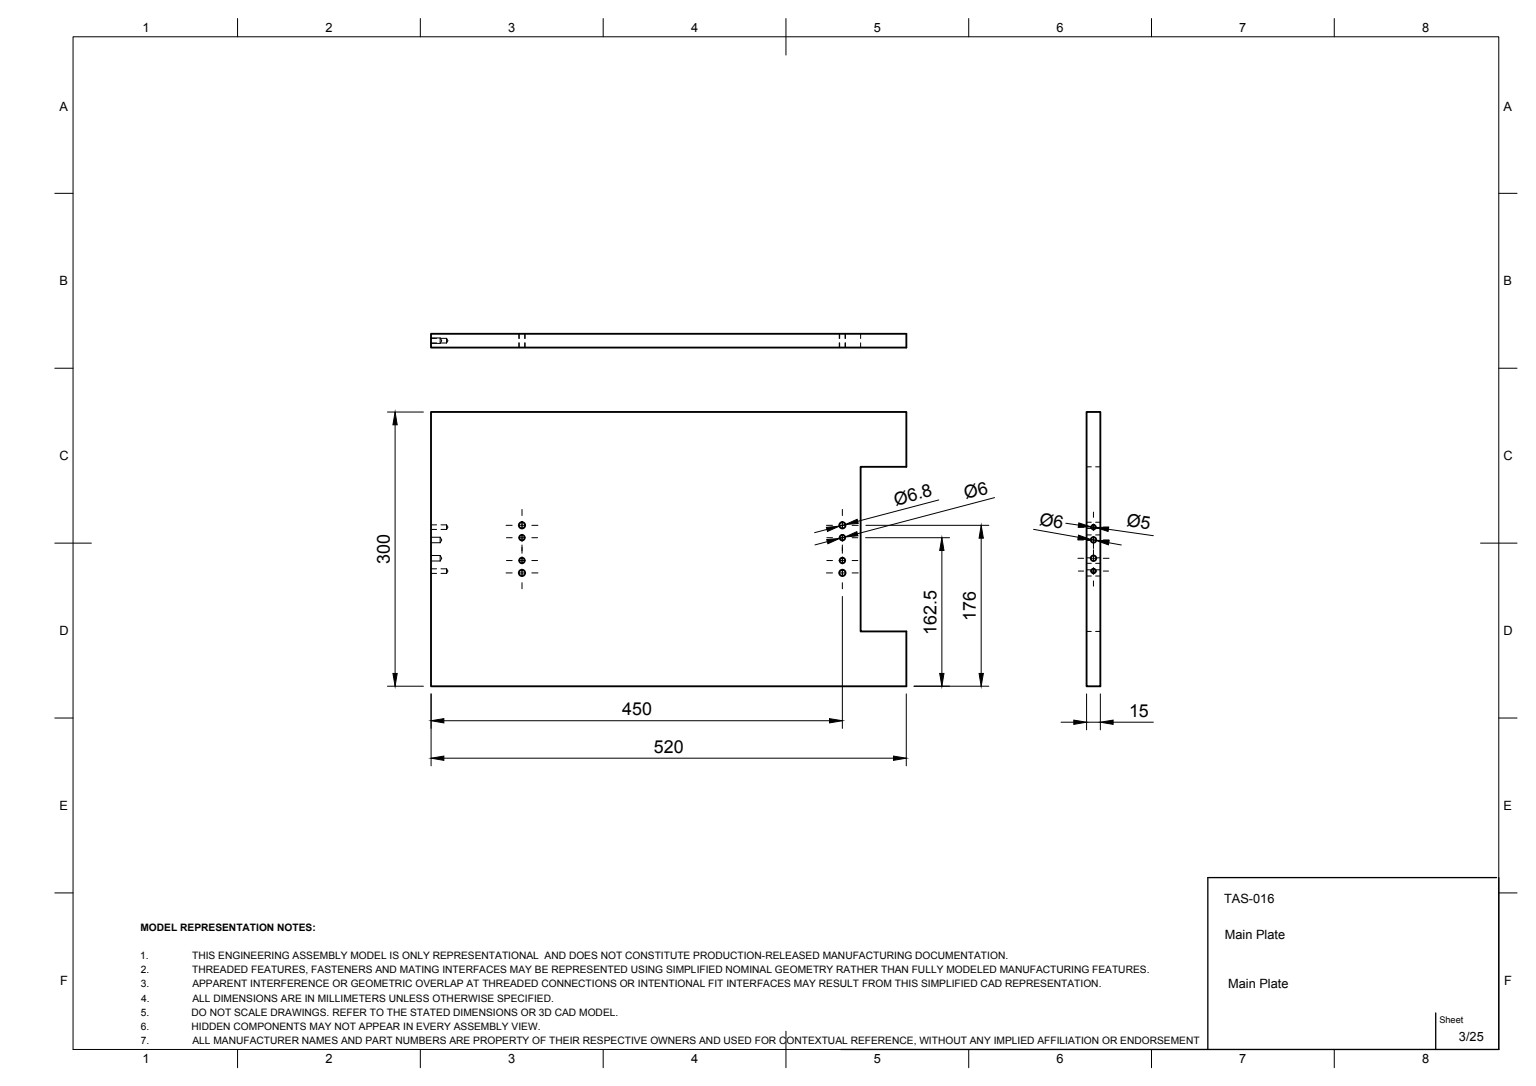
ISO-10303-21;
HEADER;
/* Generated by software containing ST-Developer
 * from STEP Tools, Inc. (www.steptools.com) 
 */

FILE_DESCRIPTION(
/* description */ ('STEP AP214'),
/* implementation_level */ '2;1');

FILE_NAME(
/* name */ 'Main Plate.step',
/* time_stamp */ '2026-11-15T14:55:55-08:00',
/* author */ (''),
/* organization */ (''),
/* preprocessor_version */ 'ST-DEVELOPER v20.2',
/* originating_system */ 'Autodesk Translation Framework v15.17.0.0',
/* authorisation */ '');

FILE_SCHEMA (('AUTOMOTIVE_DESIGN { 1 0 10303 214 3 1 1 }'));
ENDSEC;

DATA;
#10=MECHANICAL_DESIGN_GEOMETRIC_PRESENTATION_REPRESENTATION('',(#926),#57079);
#868=SHAPE_REPRESENTATION_RELATIONSHIP('SRR','None',#57250,#897);
#897=ADVANCED_BREP_SHAPE_REPRESENTATION('',(#963),#57042);
#926=STYLED_ITEM('',(#57444),#963);
#963=MANIFOLD_SOLID_BREP('Body1',#24526);
#1000=FACE_BOUND('',#3553,.T.);
#1001=FACE_BOUND('',#3554,.T.);
#1002=FACE_BOUND('',#3555,.T.);
#1003=FACE_BOUND('',#3556,.T.);
#1004=FACE_BOUND('',#3560,.T.);
#1005=FACE_BOUND('',#3561,.T.);
#1006=FACE_BOUND('',#3562,.T.);
#1007=FACE_BOUND('',#3563,.T.);
#1008=FACE_BOUND('',#3564,.T.);
#1009=FACE_BOUND('',#3565,.T.);
#1010=FACE_BOUND('',#3566,.T.);
#1011=FACE_BOUND('',#3567,.T.);
#1012=FACE_BOUND('',#3569,.T.);
#1013=FACE_BOUND('',#3570,.T.);
#1014=FACE_BOUND('',#3571,.T.);
#1015=FACE_BOUND('',#3572,.T.);
#1016=FACE_BOUND('',#3573,.T.);
#1017=FACE_BOUND('',#3574,.T.);
#1018=FACE_BOUND('',#3575,.T.);
#1019=FACE_BOUND('',#3576,.T.);
#1342=PLANE('',#24925);
#1343=PLANE('',#24926);
#1344=PLANE('',#24927);
#1345=PLANE('',#24928);
#1346=PLANE('',#24929);
#1347=PLANE('',#24930);
#1348=PLANE('',#24931);
#1349=PLANE('',#24932);
#1350=PLANE('',#24933);
#1351=PLANE('',#24934);
#2105=CONICAL_SURFACE('',#24912,3.,1.02974425867665);
#2106=CONICAL_SURFACE('',#24916,3.,1.02974425867665);
#2107=CONICAL_SURFACE('',#24920,2.49999999999999,1.02974425867666);
#2108=CONICAL_SURFACE('',#24924,2.49999999999999,1.02974425867666);
#2159=FACE_OUTER_BOUND('',#3534,.T.);
#2160=FACE_OUTER_BOUND('',#3535,.T.);
#2161=FACE_OUTER_BOUND('',#3536,.T.);
#2162=FACE_OUTER_BOUND('',#3537,.T.);
#2163=FACE_OUTER_BOUND('',#3538,.T.);
#2164=FACE_OUTER_BOUND('',#3539,.T.);
#2165=FACE_OUTER_BOUND('',#3540,.T.);
#2166=FACE_OUTER_BOUND('',#3541,.T.);
#2167=FACE_OUTER_BOUND('',#3542,.T.);
#2168=FACE_OUTER_BOUND('',#3543,.T.);
#2169=FACE_OUTER_BOUND('',#3544,.T.);
#2170=FACE_OUTER_BOUND('',#3545,.T.);
#2171=FACE_OUTER_BOUND('',#3546,.T.);
#2172=FACE_OUTER_BOUND('',#3547,.T.);
#2173=FACE_OUTER_BOUND('',#3548,.T.);
#2174=FACE_OUTER_BOUND('',#3549,.T.);
#2175=FACE_OUTER_BOUND('',#3550,.T.);
#2176=FACE_OUTER_BOUND('',#3551,.T.);
#2177=FACE_OUTER_BOUND('',#3552,.T.);
#2178=FACE_OUTER_BOUND('',#3557,.T.);
#2179=FACE_OUTER_BOUND('',#3558,.T.);
#2180=FACE_OUTER_BOUND('',#3559,.T.);
#2181=FACE_OUTER_BOUND('',#3568,.T.);
#2182=FACE_OUTER_BOUND('',#3577,.T.);
#2183=FACE_OUTER_BOUND('',#3578,.T.);
#2184=FACE_OUTER_BOUND('',#3579,.T.);
#3534=EDGE_LOOP('',(#15916,#15917,#15918,#15919));
#3535=EDGE_LOOP('',(#15920,#15921,#15922,#15923));
#3536=EDGE_LOOP('',(#15924,#15925,#15926,#15927));
#3537=EDGE_LOOP('',(#15928,#15929,#15930,#15931));
#3538=EDGE_LOOP('',(#15932,#15933,#15934,#15935));
#3539=EDGE_LOOP('',(#15936,#15937,#15938,#15939));
#3540=EDGE_LOOP('',(#15940,#15941,#15942,#15943));
#3541=EDGE_LOOP('',(#15944,#15945,#15946,#15947));
#3542=EDGE_LOOP('',(#15948,#15949,#15950,#15951));
#3543=EDGE_LOOP('',(#15952,#15953,#15954));
#3544=EDGE_LOOP('',(#15955,#15956,#15957,#15958));
#3545=EDGE_LOOP('',(#15959,#15960,#15961));
#3546=EDGE_LOOP('',(#15962,#15963,#15964,#15965));
#3547=EDGE_LOOP('',(#15966,#15967,#15968));
#3548=EDGE_LOOP('',(#15969,#15970,#15971,#15972));
#3549=EDGE_LOOP('',(#15973,#15974,#15975));
#3550=EDGE_LOOP('',(#15976,#15977,#15978,#15979));
#3551=EDGE_LOOP('',(#15980,#15981,#15982,#15983));
#3552=EDGE_LOOP('',(#15984,#15985,#15986,#15987));
#3553=EDGE_LOOP('',(#15988));
#3554=EDGE_LOOP('',(#15989));
#3555=EDGE_LOOP('',(#15990));
#3556=EDGE_LOOP('',(#15991));
#3557=EDGE_LOOP('',(#15992,#15993,#15994,#15995));
#3558=EDGE_LOOP('',(#15996,#15997,#15998,#15999));
#3559=EDGE_LOOP('',(#16000,#16001,#16002,#16003,#16004,#16005,#16006,#16007));
#3560=EDGE_LOOP('',(#16008));
#3561=EDGE_LOOP('',(#16009));
#3562=EDGE_LOOP('',(#16010));
#3563=EDGE_LOOP('',(#16011));
#3564=EDGE_LOOP('',(#16012));
#3565=EDGE_LOOP('',(#16013));
#3566=EDGE_LOOP('',(#16014));
#3567=EDGE_LOOP('',(#16015));
#3568=EDGE_LOOP('',(#16016,#16017,#16018,#16019,#16020,#16021,#16022,#16023));
#3569=EDGE_LOOP('',(#16024));
#3570=EDGE_LOOP('',(#16025));
#3571=EDGE_LOOP('',(#16026));
#3572=EDGE_LOOP('',(#16027));
#3573=EDGE_LOOP('',(#16028));
#3574=EDGE_LOOP('',(#16029));
#3575=EDGE_LOOP('',(#16030));
#3576=EDGE_LOOP('',(#16031));
#3577=EDGE_LOOP('',(#16032,#16033,#16034,#16035));
#3578=EDGE_LOOP('',(#16036,#16037,#16038,#16039));
#3579=EDGE_LOOP('',(#16040,#16041,#16042,#16043));
#5251=LINE('',#34638,#7218);
#5252=LINE('',#34644,#7219);
#5253=LINE('',#34650,#7220);
#5254=LINE('',#34656,#7221);
#5255=LINE('',#34662,#7222);
#5256=LINE('',#34668,#7223);
#5257=LINE('',#34674,#7224);
#5258=LINE('',#34680,#7225);
#5259=LINE('',#34686,#7226);
#5260=LINE('',#34690,#7227);
#5261=LINE('',#34695,#7228);
#5262=LINE('',#34699,#7229);
#5263=LINE('',#34704,#7230);
#5264=LINE('',#34708,#7231);
#5265=LINE('',#34713,#7232);
#5266=LINE('',#34717,#7233);
#5267=LINE('',#34721,#7234);
#5268=LINE('',#34723,#7235);
#5269=LINE('',#34725,#7236);
#5270=LINE('',#34726,#7237);
#5271=LINE('',#34730,#7238);
#5272=LINE('',#34732,#7239);
#5273=LINE('',#34734,#7240);
#5274=LINE('',#34735,#7241);
#5275=LINE('',#34738,#7242);
#5276=LINE('',#34740,#7243);
#5277=LINE('',#34741,#7244);
#5278=LINE('',#34743,#7245);
#5279=LINE('',#34744,#7246);
#5280=LINE('',#34747,#7247);
#5281=LINE('',#34749,#7248);
#5282=LINE('',#34750,#7249);
#5283=LINE('',#34753,#7250);
#5284=LINE('',#34755,#7251);
#5285=LINE('',#34756,#7252);
#5286=LINE('',#34759,#7253);
#5287=LINE('',#34761,#7254);
#5288=LINE('',#34762,#7255);
#5289=LINE('',#34764,#7256);
#5290=LINE('',#34766,#7257);
#7218=VECTOR('',#27485,3.);
#7219=VECTOR('',#27492,3.);
#7220=VECTOR('',#27499,3.);
#7221=VECTOR('',#27506,3.);
#7222=VECTOR('',#27513,3.4);
#7223=VECTOR('',#27520,3.4);
#7224=VECTOR('',#27527,3.4);
#7225=VECTOR('',#27534,3.4);
#7226=VECTOR('',#27541,3.);
#7227=VECTOR('',#27546,3.);
#7228=VECTOR('',#27551,3.);
#7229=VECTOR('',#27556,3.);
#7230=VECTOR('',#27561,2.49999999999999);
#7231=VECTOR('',#27566,2.49999999999999);
#7232=VECTOR('',#27571,2.49999999999999);
#7233=VECTOR('',#27576,2.49999999999999);
#7234=VECTOR('',#27579,1000.);
#7235=VECTOR('',#27580,1000.);
#7236=VECTOR('',#27581,1000.);
#7237=VECTOR('',#27582,1000.);
#7238=VECTOR('',#27585,1000.);
#7239=VECTOR('',#27586,1000.);
#7240=VECTOR('',#27587,1000.);
#7241=VECTOR('',#27588,1000.);
#7242=VECTOR('',#27591,1000.);
#7243=VECTOR('',#27592,1000.);
#7244=VECTOR('',#27593,1000.);
#7245=VECTOR('',#27596,1000.);
#7246=VECTOR('',#27597,1000.);
#7247=VECTOR('',#27600,1000.);
#7248=VECTOR('',#27601,1000.);
#7249=VECTOR('',#27602,1000.);
#7250=VECTOR('',#27605,1000.);
#7251=VECTOR('',#27606,1000.);
#7252=VECTOR('',#27607,1000.);
#7253=VECTOR('',#27610,1000.);
#7254=VECTOR('',#27611,1000.);
#7255=VECTOR('',#27612,1000.);
#7256=VECTOR('',#27615,1000.);
#7257=VECTOR('',#27618,1000.);
#9185=CIRCLE('',#24886,3.);
#9186=CIRCLE('',#24887,3.);
#9187=CIRCLE('',#24889,3.);
#9188=CIRCLE('',#24890,3.);
#9189=CIRCLE('',#24892,3.);
#9190=CIRCLE('',#24893,3.);
#9191=CIRCLE('',#24895,3.);
#9192=CIRCLE('',#24896,3.);
#9193=CIRCLE('',#24898,3.4);
#9194=CIRCLE('',#24899,3.4);
#9195=CIRCLE('',#24901,3.4);
#9196=CIRCLE('',#24902,3.4);
#9197=CIRCLE('',#24904,3.4);
#9198=CIRCLE('',#24905,3.4);
#9199=CIRCLE('',#24907,3.4);
#9200=CIRCLE('',#24908,3.4);
#9201=CIRCLE('',#24910,3.);
#9202=CIRCLE('',#24911,3.);
#9203=CIRCLE('',#24914,3.);
#9204=CIRCLE('',#24915,3.);
#9205=CIRCLE('',#24918,2.49999999999999);
#9206=CIRCLE('',#24919,2.49999999999999);
#9207=CIRCLE('',#24922,2.49999999999999);
#9208=CIRCLE('',#24923,2.49999999999999);
#10279=VERTEX_POINT('',#34635);
#10280=VERTEX_POINT('',#34637);
#10281=VERTEX_POINT('',#34641);
#10282=VERTEX_POINT('',#34643);
#10283=VERTEX_POINT('',#34647);
#10284=VERTEX_POINT('',#34649);
#10285=VERTEX_POINT('',#34653);
#10286=VERTEX_POINT('',#34655);
#10287=VERTEX_POINT('',#34659);
#10288=VERTEX_POINT('',#34661);
#10289=VERTEX_POINT('',#34665);
#10290=VERTEX_POINT('',#34667);
#10291=VERTEX_POINT('',#34671);
#10292=VERTEX_POINT('',#34673);
#10293=VERTEX_POINT('',#34677);
#10294=VERTEX_POINT('',#34679);
#10295=VERTEX_POINT('',#34683);
#10296=VERTEX_POINT('',#34685);
#10297=VERTEX_POINT('',#34689);
#10298=VERTEX_POINT('',#34692);
#10299=VERTEX_POINT('',#34694);
#10300=VERTEX_POINT('',#34698);
#10301=VERTEX_POINT('',#34701);
#10302=VERTEX_POINT('',#34703);
#10303=VERTEX_POINT('',#34707);
#10304=VERTEX_POINT('',#34710);
#10305=VERTEX_POINT('',#34712);
#10306=VERTEX_POINT('',#34716);
#10307=VERTEX_POINT('',#34719);
#10308=VERTEX_POINT('',#34720);
#10309=VERTEX_POINT('',#34722);
#10310=VERTEX_POINT('',#34724);
#10311=VERTEX_POINT('',#34728);
#10312=VERTEX_POINT('',#34729);
#10313=VERTEX_POINT('',#34731);
#10314=VERTEX_POINT('',#34733);
#10315=VERTEX_POINT('',#34737);
#10316=VERTEX_POINT('',#34739);
#10317=VERTEX_POINT('',#34746);
#10318=VERTEX_POINT('',#34748);
#10319=VERTEX_POINT('',#34752);
#10320=VERTEX_POINT('',#34754);
#10321=VERTEX_POINT('',#34758);
#10322=VERTEX_POINT('',#34760);
#12503=EDGE_CURVE('',#10279,#10279,#9185,.T.);
#12504=EDGE_CURVE('',#10279,#10280,#5251,.T.);
#12505=EDGE_CURVE('',#10280,#10280,#9186,.T.);
#12506=EDGE_CURVE('',#10281,#10281,#9187,.T.);
#12507=EDGE_CURVE('',#10281,#10282,#5252,.T.);
#12508=EDGE_CURVE('',#10282,#10282,#9188,.T.);
#12509=EDGE_CURVE('',#10283,#10283,#9189,.T.);
#12510=EDGE_CURVE('',#10283,#10284,#5253,.T.);
#12511=EDGE_CURVE('',#10284,#10284,#9190,.T.);
#12512=EDGE_CURVE('',#10285,#10285,#9191,.T.);
#12513=EDGE_CURVE('',#10285,#10286,#5254,.T.);
#12514=EDGE_CURVE('',#10286,#10286,#9192,.T.);
#12515=EDGE_CURVE('',#10287,#10287,#9193,.T.);
#12516=EDGE_CURVE('',#10287,#10288,#5255,.T.);
#12517=EDGE_CURVE('',#10288,#10288,#9194,.T.);
#12518=EDGE_CURVE('',#10289,#10289,#9195,.T.);
#12519=EDGE_CURVE('',#10289,#10290,#5256,.T.);
#12520=EDGE_CURVE('',#10290,#10290,#9196,.T.);
#12521=EDGE_CURVE('',#10291,#10291,#9197,.T.);
#12522=EDGE_CURVE('',#10291,#10292,#5257,.T.);
#12523=EDGE_CURVE('',#10292,#10292,#9198,.T.);
#12524=EDGE_CURVE('',#10293,#10293,#9199,.T.);
#12525=EDGE_CURVE('',#10293,#10294,#5258,.T.);
#12526=EDGE_CURVE('',#10294,#10294,#9200,.T.);
#12527=EDGE_CURVE('',#10295,#10295,#9201,.T.);
#12528=EDGE_CURVE('',#10295,#10296,#5259,.T.);
#12529=EDGE_CURVE('',#10296,#10296,#9202,.T.);
#12530=EDGE_CURVE('',#10297,#10295,#5260,.T.);
#12531=EDGE_CURVE('',#10298,#10298,#9203,.T.);
#12532=EDGE_CURVE('',#10298,#10299,#5261,.T.);
#12533=EDGE_CURVE('',#10299,#10299,#9204,.T.);
#12534=EDGE_CURVE('',#10300,#10298,#5262,.T.);
#12535=EDGE_CURVE('',#10301,#10301,#9205,.T.);
#12536=EDGE_CURVE('',#10301,#10302,#5263,.T.);
#12537=EDGE_CURVE('',#10302,#10302,#9206,.T.);
#12538=EDGE_CURVE('',#10303,#10301,#5264,.T.);
#12539=EDGE_CURVE('',#10304,#10304,#9207,.T.);
#12540=EDGE_CURVE('',#10304,#10305,#5265,.T.);
#12541=EDGE_CURVE('',#10305,#10305,#9208,.T.);
#12542=EDGE_CURVE('',#10306,#10304,#5266,.T.);
#12543=EDGE_CURVE('',#10307,#10308,#5267,.T.);
#12544=EDGE_CURVE('',#10308,#10309,#5268,.T.);
#12545=EDGE_CURVE('',#10310,#10309,#5269,.T.);
#12546=EDGE_CURVE('',#10310,#10307,#5270,.T.);
#12547=EDGE_CURVE('',#10311,#10312,#5271,.T.);
#12548=EDGE_CURVE('',#10313,#10312,#5272,.T.);
#12549=EDGE_CURVE('',#10314,#10313,#5273,.T.);
#12550=EDGE_CURVE('',#10314,#10311,#5274,.T.);
#12551=EDGE_CURVE('',#10312,#10315,#5275,.T.);
#12552=EDGE_CURVE('',#10316,#10315,#5276,.T.);
#12553=EDGE_CURVE('',#10313,#10316,#5277,.T.);
#12554=EDGE_CURVE('',#10315,#10307,#5278,.T.);
#12555=EDGE_CURVE('',#10316,#10310,#5279,.T.);
#12556=EDGE_CURVE('',#10317,#10314,#5280,.T.);
#12557=EDGE_CURVE('',#10318,#10317,#5281,.T.);
#12558=EDGE_CURVE('',#10318,#10311,#5282,.T.);
#12559=EDGE_CURVE('',#10319,#10309,#5283,.T.);
#12560=EDGE_CURVE('',#10320,#10319,#5284,.T.);
#12561=EDGE_CURVE('',#10317,#10320,#5285,.T.);
#12562=EDGE_CURVE('',#10321,#10308,#5286,.T.);
#12563=EDGE_CURVE('',#10318,#10322,#5287,.T.);
#12564=EDGE_CURVE('',#10322,#10321,#5288,.T.);
#12565=EDGE_CURVE('',#10321,#10319,#5289,.T.);
#12566=EDGE_CURVE('',#10322,#10320,#5290,.T.);
#15916=ORIENTED_EDGE('',*,*,#12503,.F.);
#15917=ORIENTED_EDGE('',*,*,#12504,.T.);
#15918=ORIENTED_EDGE('',*,*,#12505,.T.);
#15919=ORIENTED_EDGE('',*,*,#12504,.F.);
#15920=ORIENTED_EDGE('',*,*,#12506,.F.);
#15921=ORIENTED_EDGE('',*,*,#12507,.T.);
#15922=ORIENTED_EDGE('',*,*,#12508,.T.);
#15923=ORIENTED_EDGE('',*,*,#12507,.F.);
#15924=ORIENTED_EDGE('',*,*,#12509,.F.);
#15925=ORIENTED_EDGE('',*,*,#12510,.T.);
#15926=ORIENTED_EDGE('',*,*,#12511,.T.);
#15927=ORIENTED_EDGE('',*,*,#12510,.F.);
#15928=ORIENTED_EDGE('',*,*,#12512,.F.);
#15929=ORIENTED_EDGE('',*,*,#12513,.T.);
#15930=ORIENTED_EDGE('',*,*,#12514,.T.);
#15931=ORIENTED_EDGE('',*,*,#12513,.F.);
#15932=ORIENTED_EDGE('',*,*,#12515,.F.);
#15933=ORIENTED_EDGE('',*,*,#12516,.T.);
#15934=ORIENTED_EDGE('',*,*,#12517,.T.);
#15935=ORIENTED_EDGE('',*,*,#12516,.F.);
#15936=ORIENTED_EDGE('',*,*,#12518,.F.);
#15937=ORIENTED_EDGE('',*,*,#12519,.T.);
#15938=ORIENTED_EDGE('',*,*,#12520,.T.);
#15939=ORIENTED_EDGE('',*,*,#12519,.F.);
#15940=ORIENTED_EDGE('',*,*,#12521,.F.);
#15941=ORIENTED_EDGE('',*,*,#12522,.T.);
#15942=ORIENTED_EDGE('',*,*,#12523,.T.);
#15943=ORIENTED_EDGE('',*,*,#12522,.F.);
#15944=ORIENTED_EDGE('',*,*,#12524,.F.);
#15945=ORIENTED_EDGE('',*,*,#12525,.T.);
#15946=ORIENTED_EDGE('',*,*,#12526,.T.);
#15947=ORIENTED_EDGE('',*,*,#12525,.F.);
#15948=ORIENTED_EDGE('',*,*,#12527,.F.);
#15949=ORIENTED_EDGE('',*,*,#12528,.T.);
#15950=ORIENTED_EDGE('',*,*,#12529,.T.);
#15951=ORIENTED_EDGE('',*,*,#12528,.F.);
#15952=ORIENTED_EDGE('',*,*,#12530,.T.);
#15953=ORIENTED_EDGE('',*,*,#12527,.T.);
#15954=ORIENTED_EDGE('',*,*,#12530,.F.);
#15955=ORIENTED_EDGE('',*,*,#12531,.F.);
#15956=ORIENTED_EDGE('',*,*,#12532,.T.);
#15957=ORIENTED_EDGE('',*,*,#12533,.T.);
#15958=ORIENTED_EDGE('',*,*,#12532,.F.);
#15959=ORIENTED_EDGE('',*,*,#12534,.T.);
#15960=ORIENTED_EDGE('',*,*,#12531,.T.);
#15961=ORIENTED_EDGE('',*,*,#12534,.F.);
#15962=ORIENTED_EDGE('',*,*,#12535,.F.);
#15963=ORIENTED_EDGE('',*,*,#12536,.T.);
#15964=ORIENTED_EDGE('',*,*,#12537,.T.);
#15965=ORIENTED_EDGE('',*,*,#12536,.F.);
#15966=ORIENTED_EDGE('',*,*,#12538,.T.);
#15967=ORIENTED_EDGE('',*,*,#12535,.T.);
#15968=ORIENTED_EDGE('',*,*,#12538,.F.);
#15969=ORIENTED_EDGE('',*,*,#12539,.F.);
#15970=ORIENTED_EDGE('',*,*,#12540,.T.);
#15971=ORIENTED_EDGE('',*,*,#12541,.T.);
#15972=ORIENTED_EDGE('',*,*,#12540,.F.);
#15973=ORIENTED_EDGE('',*,*,#12542,.T.);
#15974=ORIENTED_EDGE('',*,*,#12539,.T.);
#15975=ORIENTED_EDGE('',*,*,#12542,.F.);
#15976=ORIENTED_EDGE('',*,*,#12543,.T.);
#15977=ORIENTED_EDGE('',*,*,#12544,.T.);
#15978=ORIENTED_EDGE('',*,*,#12545,.F.);
#15979=ORIENTED_EDGE('',*,*,#12546,.T.);
#15980=ORIENTED_EDGE('',*,*,#12547,.T.);
#15981=ORIENTED_EDGE('',*,*,#12548,.F.);
#15982=ORIENTED_EDGE('',*,*,#12549,.F.);
#15983=ORIENTED_EDGE('',*,*,#12550,.T.);
#15984=ORIENTED_EDGE('',*,*,#12551,.T.);
#15985=ORIENTED_EDGE('',*,*,#12552,.F.);
#15986=ORIENTED_EDGE('',*,*,#12553,.F.);
#15987=ORIENTED_EDGE('',*,*,#12548,.T.);
#15988=ORIENTED_EDGE('',*,*,#12529,.F.);
#15989=ORIENTED_EDGE('',*,*,#12533,.F.);
#15990=ORIENTED_EDGE('',*,*,#12537,.F.);
#15991=ORIENTED_EDGE('',*,*,#12541,.F.);
#15992=ORIENTED_EDGE('',*,*,#12554,.T.);
#15993=ORIENTED_EDGE('',*,*,#12546,.F.);
#15994=ORIENTED_EDGE('',*,*,#12555,.F.);
#15995=ORIENTED_EDGE('',*,*,#12552,.T.);
#15996=ORIENTED_EDGE('',*,*,#12556,.F.);
#15997=ORIENTED_EDGE('',*,*,#12557,.F.);
#15998=ORIENTED_EDGE('',*,*,#12558,.T.);
#15999=ORIENTED_EDGE('',*,*,#12550,.F.);
#16000=ORIENTED_EDGE('',*,*,#12545,.T.);
#16001=ORIENTED_EDGE('',*,*,#12559,.F.);
#16002=ORIENTED_EDGE('',*,*,#12560,.F.);
#16003=ORIENTED_EDGE('',*,*,#12561,.F.);
#16004=ORIENTED_EDGE('',*,*,#12556,.T.);
#16005=ORIENTED_EDGE('',*,*,#12549,.T.);
#16006=ORIENTED_EDGE('',*,*,#12553,.T.);
#16007=ORIENTED_EDGE('',*,*,#12555,.T.);
#16008=ORIENTED_EDGE('',*,*,#12505,.F.);
#16009=ORIENTED_EDGE('',*,*,#12508,.F.);
#16010=ORIENTED_EDGE('',*,*,#12511,.F.);
#16011=ORIENTED_EDGE('',*,*,#12514,.F.);
#16012=ORIENTED_EDGE('',*,*,#12517,.F.);
#16013=ORIENTED_EDGE('',*,*,#12520,.F.);
#16014=ORIENTED_EDGE('',*,*,#12523,.F.);
#16015=ORIENTED_EDGE('',*,*,#12526,.F.);
#16016=ORIENTED_EDGE('',*,*,#12562,.T.);
#16017=ORIENTED_EDGE('',*,*,#12543,.F.);
#16018=ORIENTED_EDGE('',*,*,#12554,.F.);
#16019=ORIENTED_EDGE('',*,*,#12551,.F.);
#16020=ORIENTED_EDGE('',*,*,#12547,.F.);
#16021=ORIENTED_EDGE('',*,*,#12558,.F.);
#16022=ORIENTED_EDGE('',*,*,#12563,.T.);
#16023=ORIENTED_EDGE('',*,*,#12564,.T.);
#16024=ORIENTED_EDGE('',*,*,#12503,.T.);
#16025=ORIENTED_EDGE('',*,*,#12506,.T.);
#16026=ORIENTED_EDGE('',*,*,#12509,.T.);
#16027=ORIENTED_EDGE('',*,*,#12512,.T.);
#16028=ORIENTED_EDGE('',*,*,#12515,.T.);
#16029=ORIENTED_EDGE('',*,*,#12518,.T.);
#16030=ORIENTED_EDGE('',*,*,#12521,.T.);
#16031=ORIENTED_EDGE('',*,*,#12524,.T.);
#16032=ORIENTED_EDGE('',*,*,#12559,.T.);
#16033=ORIENTED_EDGE('',*,*,#12544,.F.);
#16034=ORIENTED_EDGE('',*,*,#12562,.F.);
#16035=ORIENTED_EDGE('',*,*,#12565,.T.);
#16036=ORIENTED_EDGE('',*,*,#12560,.T.);
#16037=ORIENTED_EDGE('',*,*,#12565,.F.);
#16038=ORIENTED_EDGE('',*,*,#12564,.F.);
#16039=ORIENTED_EDGE('',*,*,#12566,.T.);
#16040=ORIENTED_EDGE('',*,*,#12561,.T.);
#16041=ORIENTED_EDGE('',*,*,#12566,.F.);
#16042=ORIENTED_EDGE('',*,*,#12563,.F.);
#16043=ORIENTED_EDGE('',*,*,#12557,.T.);
#22742=CYLINDRICAL_SURFACE('',#24885,3.);
#22743=CYLINDRICAL_SURFACE('',#24888,3.);
#22744=CYLINDRICAL_SURFACE('',#24891,3.);
#22745=CYLINDRICAL_SURFACE('',#24894,3.);
#22746=CYLINDRICAL_SURFACE('',#24897,3.4);
#22747=CYLINDRICAL_SURFACE('',#24900,3.4);
#22748=CYLINDRICAL_SURFACE('',#24903,3.4);
#22749=CYLINDRICAL_SURFACE('',#24906,3.4);
#22750=CYLINDRICAL_SURFACE('',#24909,3.);
#22751=CYLINDRICAL_SURFACE('',#24913,3.);
#22752=CYLINDRICAL_SURFACE('',#24917,2.49999999999999);
#22753=CYLINDRICAL_SURFACE('',#24921,2.49999999999999);
#23151=ADVANCED_FACE('',(#2159),#22742,.F.);
#23152=ADVANCED_FACE('',(#2160),#22743,.F.);
#23153=ADVANCED_FACE('',(#2161),#22744,.F.);
#23154=ADVANCED_FACE('',(#2162),#22745,.F.);
#23155=ADVANCED_FACE('',(#2163),#22746,.F.);
#23156=ADVANCED_FACE('',(#2164),#22747,.F.);
#23157=ADVANCED_FACE('',(#2165),#22748,.F.);
#23158=ADVANCED_FACE('',(#2166),#22749,.F.);
#23159=ADVANCED_FACE('',(#2167),#22750,.F.);
#23160=ADVANCED_FACE('',(#2168),#2105,.F.);
#23161=ADVANCED_FACE('',(#2169),#22751,.F.);
#23162=ADVANCED_FACE('',(#2170),#2106,.F.);
#23163=ADVANCED_FACE('',(#2171),#22752,.F.);
#23164=ADVANCED_FACE('',(#2172),#2107,.F.);
#23165=ADVANCED_FACE('',(#2173),#22753,.F.);
#23166=ADVANCED_FACE('',(#2174),#2108,.F.);
#23167=ADVANCED_FACE('',(#2175),#1342,.F.);
#23168=ADVANCED_FACE('',(#2176),#1343,.F.);
#23169=ADVANCED_FACE('',(#2177,#1000,#1001,#1002,#1003),#1344,.F.);
#23170=ADVANCED_FACE('',(#2178),#1345,.F.);
#23171=ADVANCED_FACE('',(#2179),#1346,.F.);
#23172=ADVANCED_FACE('',(#2180,#1004,#1005,#1006,#1007,#1008,#1009,#1010,
#1011),#1347,.F.);
#23173=ADVANCED_FACE('',(#2181,#1012,#1013,#1014,#1015,#1016,#1017,#1018,
#1019),#1348,.T.);
#23174=ADVANCED_FACE('',(#2182),#1349,.F.);
#23175=ADVANCED_FACE('',(#2183),#1350,.F.);
#23176=ADVANCED_FACE('',(#2184),#1351,.F.);
#24526=CLOSED_SHELL('',(#23151,#23152,#23153,#23154,#23155,#23156,#23157,
#23158,#23159,#23160,#23161,#23162,#23163,#23164,#23165,#23166,#23167,#23168,
#23169,#23170,#23171,#23172,#23173,#23174,#23175,#23176));
#24884=AXIS2_PLACEMENT_3D('',#34633,#27479,#27480);
#24885=AXIS2_PLACEMENT_3D('',#34634,#27481,#27482);
#24886=AXIS2_PLACEMENT_3D('',#34636,#27483,#27484);
#24887=AXIS2_PLACEMENT_3D('',#34639,#27486,#27487);
#24888=AXIS2_PLACEMENT_3D('',#34640,#27488,#27489);
#24889=AXIS2_PLACEMENT_3D('',#34642,#27490,#27491);
#24890=AXIS2_PLACEMENT_3D('',#34645,#27493,#27494);
#24891=AXIS2_PLACEMENT_3D('',#34646,#27495,#27496);
#24892=AXIS2_PLACEMENT_3D('',#34648,#27497,#27498);
#24893=AXIS2_PLACEMENT_3D('',#34651,#27500,#27501);
#24894=AXIS2_PLACEMENT_3D('',#34652,#27502,#27503);
#24895=AXIS2_PLACEMENT_3D('',#34654,#27504,#27505);
#24896=AXIS2_PLACEMENT_3D('',#34657,#27507,#27508);
#24897=AXIS2_PLACEMENT_3D('',#34658,#27509,#27510);
#24898=AXIS2_PLACEMENT_3D('',#34660,#27511,#27512);
#24899=AXIS2_PLACEMENT_3D('',#34663,#27514,#27515);
#24900=AXIS2_PLACEMENT_3D('',#34664,#27516,#27517);
#24901=AXIS2_PLACEMENT_3D('',#34666,#27518,#27519);
#24902=AXIS2_PLACEMENT_3D('',#34669,#27521,#27522);
#24903=AXIS2_PLACEMENT_3D('',#34670,#27523,#27524);
#24904=AXIS2_PLACEMENT_3D('',#34672,#27525,#27526);
#24905=AXIS2_PLACEMENT_3D('',#34675,#27528,#27529);
#24906=AXIS2_PLACEMENT_3D('',#34676,#27530,#27531);
#24907=AXIS2_PLACEMENT_3D('',#34678,#27532,#27533);
#24908=AXIS2_PLACEMENT_3D('',#34681,#27535,#27536);
#24909=AXIS2_PLACEMENT_3D('',#34682,#27537,#27538);
#24910=AXIS2_PLACEMENT_3D('',#34684,#27539,#27540);
#24911=AXIS2_PLACEMENT_3D('',#34687,#27542,#27543);
#24912=AXIS2_PLACEMENT_3D('',#34688,#27544,#27545);
#24913=AXIS2_PLACEMENT_3D('',#34691,#27547,#27548);
#24914=AXIS2_PLACEMENT_3D('',#34693,#27549,#27550);
#24915=AXIS2_PLACEMENT_3D('',#34696,#27552,#27553);
#24916=AXIS2_PLACEMENT_3D('',#34697,#27554,#27555);
#24917=AXIS2_PLACEMENT_3D('',#34700,#27557,#27558);
#24918=AXIS2_PLACEMENT_3D('',#34702,#27559,#27560);
#24919=AXIS2_PLACEMENT_3D('',#34705,#27562,#27563);
#24920=AXIS2_PLACEMENT_3D('',#34706,#27564,#27565);
#24921=AXIS2_PLACEMENT_3D('',#34709,#27567,#27568);
#24922=AXIS2_PLACEMENT_3D('',#34711,#27569,#27570);
#24923=AXIS2_PLACEMENT_3D('',#34714,#27572,#27573);
#24924=AXIS2_PLACEMENT_3D('',#34715,#27574,#27575);
#24925=AXIS2_PLACEMENT_3D('',#34718,#27577,#27578);
#24926=AXIS2_PLACEMENT_3D('',#34727,#27583,#27584);
#24927=AXIS2_PLACEMENT_3D('',#34736,#27589,#27590);
#24928=AXIS2_PLACEMENT_3D('',#34742,#27594,#27595);
#24929=AXIS2_PLACEMENT_3D('',#34745,#27598,#27599);
#24930=AXIS2_PLACEMENT_3D('',#34751,#27603,#27604);
#24931=AXIS2_PLACEMENT_3D('',#34757,#27608,#27609);
#24932=AXIS2_PLACEMENT_3D('',#34763,#27613,#27614);
#24933=AXIS2_PLACEMENT_3D('',#34765,#27616,#27617);
#24934=AXIS2_PLACEMENT_3D('',#34767,#27619,#27620);
#27479=DIRECTION('axis',(0.,0.,1.));
#27480=DIRECTION('refdir',(1.,0.,0.));
#27481=DIRECTION('center_axis',(0.,0.,1.));
#27482=DIRECTION('ref_axis',(1.,0.,0.));
#27483=DIRECTION('center_axis',(0.,0.,1.));
#27484=DIRECTION('ref_axis',(1.,0.,0.));
#27485=DIRECTION('',(0.,0.,1.));
#27486=DIRECTION('center_axis',(0.,0.,1.));
#27487=DIRECTION('ref_axis',(1.,0.,0.));
#27488=DIRECTION('center_axis',(0.,0.,1.));
#27489=DIRECTION('ref_axis',(1.,0.,0.));
#27490=DIRECTION('center_axis',(0.,0.,1.));
#27491=DIRECTION('ref_axis',(1.,0.,0.));
#27492=DIRECTION('',(0.,0.,1.));
#27493=DIRECTION('center_axis',(0.,0.,1.));
#27494=DIRECTION('ref_axis',(1.,0.,0.));
#27495=DIRECTION('center_axis',(0.,0.,1.));
#27496=DIRECTION('ref_axis',(1.,0.,0.));
#27497=DIRECTION('center_axis',(0.,0.,1.));
#27498=DIRECTION('ref_axis',(1.,0.,0.));
#27499=DIRECTION('',(0.,0.,1.));
#27500=DIRECTION('center_axis',(0.,0.,1.));
#27501=DIRECTION('ref_axis',(1.,0.,0.));
#27502=DIRECTION('center_axis',(0.,0.,1.));
#27503=DIRECTION('ref_axis',(1.,0.,0.));
#27504=DIRECTION('center_axis',(0.,0.,1.));
#27505=DIRECTION('ref_axis',(1.,0.,0.));
#27506=DIRECTION('',(0.,0.,1.));
#27507=DIRECTION('center_axis',(0.,0.,1.));
#27508=DIRECTION('ref_axis',(1.,0.,0.));
#27509=DIRECTION('center_axis',(0.,0.,1.));
#27510=DIRECTION('ref_axis',(1.,0.,0.));
#27511=DIRECTION('center_axis',(0.,0.,1.));
#27512=DIRECTION('ref_axis',(1.,0.,0.));
#27513=DIRECTION('',(0.,0.,1.));
#27514=DIRECTION('center_axis',(0.,0.,1.));
#27515=DIRECTION('ref_axis',(1.,0.,0.));
#27516=DIRECTION('center_axis',(0.,0.,1.));
#27517=DIRECTION('ref_axis',(1.,0.,0.));
#27518=DIRECTION('center_axis',(0.,0.,1.));
#27519=DIRECTION('ref_axis',(1.,0.,0.));
#27520=DIRECTION('',(0.,0.,1.));
#27521=DIRECTION('center_axis',(0.,0.,1.));
#27522=DIRECTION('ref_axis',(1.,0.,0.));
#27523=DIRECTION('center_axis',(0.,0.,1.));
#27524=DIRECTION('ref_axis',(1.,0.,0.));
#27525=DIRECTION('center_axis',(0.,0.,1.));
#27526=DIRECTION('ref_axis',(1.,0.,0.));
#27527=DIRECTION('',(0.,0.,1.));
#27528=DIRECTION('center_axis',(0.,0.,1.));
#27529=DIRECTION('ref_axis',(1.,0.,0.));
#27530=DIRECTION('center_axis',(0.,0.,1.));
#27531=DIRECTION('ref_axis',(1.,0.,0.));
#27532=DIRECTION('center_axis',(0.,0.,1.));
#27533=DIRECTION('ref_axis',(1.,0.,0.));
#27534=DIRECTION('',(0.,0.,1.));
#27535=DIRECTION('center_axis',(0.,0.,1.));
#27536=DIRECTION('ref_axis',(1.,0.,0.));
#27537=DIRECTION('center_axis',(0.,1.,0.));
#27538=DIRECTION('ref_axis',(0.,0.,1.));
#27539=DIRECTION('center_axis',(0.,1.,0.));
#27540=DIRECTION('ref_axis',(0.,0.,1.));
#27541=DIRECTION('',(0.,1.,0.));
#27542=DIRECTION('center_axis',(0.,1.,0.));
#27543=DIRECTION('ref_axis',(0.,0.,1.));
#27544=DIRECTION('center_axis',(0.,1.,0.));
#27545=DIRECTION('ref_axis',(0.,0.,1.));
#27546=DIRECTION('',(-1.04972719113862E-16,0.515038074910055,-0.857167300702112));
#27547=DIRECTION('center_axis',(0.,1.,0.));
#27548=DIRECTION('ref_axis',(0.,0.,1.));
#27549=DIRECTION('center_axis',(0.,1.,0.));
#27550=DIRECTION('ref_axis',(0.,0.,1.));
#27551=DIRECTION('',(0.,1.,0.));
#27552=DIRECTION('center_axis',(0.,1.,0.));
#27553=DIRECTION('ref_axis',(0.,0.,1.));
#27554=DIRECTION('center_axis',(0.,1.,0.));
#27555=DIRECTION('ref_axis',(0.,0.,1.));
#27556=DIRECTION('',(-1.04972719113862E-16,0.515038074910055,-0.857167300702112));
#27557=DIRECTION('center_axis',(0.,1.,0.));
#27558=DIRECTION('ref_axis',(0.,0.,1.));
#27559=DIRECTION('center_axis',(0.,1.,0.));
#27560=DIRECTION('ref_axis',(0.,0.,1.));
#27561=DIRECTION('',(0.,1.,0.));
#27562=DIRECTION('center_axis',(0.,1.,0.));
#27563=DIRECTION('ref_axis',(0.,0.,1.));
#27564=DIRECTION('center_axis',(0.,1.,0.));
#27565=DIRECTION('ref_axis',(0.,0.,1.));
#27566=DIRECTION('',(-1.04972719113862E-16,0.515038074910053,-0.857167300702113));
#27567=DIRECTION('center_axis',(0.,1.,0.));
#27568=DIRECTION('ref_axis',(0.,0.,1.));
#27569=DIRECTION('center_axis',(0.,1.,0.));
#27570=DIRECTION('ref_axis',(0.,0.,1.));
#27571=DIRECTION('',(0.,1.,0.));
#27572=DIRECTION('center_axis',(0.,1.,0.));
#27573=DIRECTION('ref_axis',(0.,0.,1.));
#27574=DIRECTION('center_axis',(0.,1.,0.));
#27575=DIRECTION('ref_axis',(0.,0.,1.));
#27576=DIRECTION('',(-1.04972719113862E-16,0.515038074910053,-0.857167300702113));
#27577=DIRECTION('center_axis',(0.,1.,0.));
#27578=DIRECTION('ref_axis',(0.,0.,1.));
#27579=DIRECTION('',(1.,0.,0.));
#27580=DIRECTION('',(0.,0.,1.));
#27581=DIRECTION('',(1.,0.,0.));
#27582=DIRECTION('',(0.,0.,-1.));
#27583=DIRECTION('center_axis',(-1.,0.,0.));
#27584=DIRECTION('ref_axis',(0.,0.,1.));
#27585=DIRECTION('',(0.,1.,0.));
#27586=DIRECTION('',(0.,0.,-1.));
#27587=DIRECTION('',(0.,1.,0.));
#27588=DIRECTION('',(0.,0.,-1.));
#27589=DIRECTION('center_axis',(0.,-1.,0.));
#27590=DIRECTION('ref_axis',(0.,0.,-1.));
#27591=DIRECTION('',(-1.,0.,0.));
#27592=DIRECTION('',(0.,0.,-1.));
#27593=DIRECTION('',(-1.,0.,0.));
#27594=DIRECTION('center_axis',(1.,0.,0.));
#27595=DIRECTION('ref_axis',(0.,0.,-1.));
#27596=DIRECTION('',(0.,-1.,0.));
#27597=DIRECTION('',(0.,-1.,0.));
#27598=DIRECTION('center_axis',(0.,1.,0.));
#27599=DIRECTION('ref_axis',(0.,0.,1.));
#27600=DIRECTION('',(1.,0.,0.));
#27601=DIRECTION('',(0.,0.,1.));
#27602=DIRECTION('',(1.,0.,0.));
#27603=DIRECTION('center_axis',(0.,0.,-1.));
#27604=DIRECTION('ref_axis',(-1.,0.,0.));
#27605=DIRECTION('',(0.,-1.,0.));
#27606=DIRECTION('',(-1.,0.,0.));
#27607=DIRECTION('',(0.,1.,0.));
#27608=DIRECTION('center_axis',(0.,0.,-1.));
#27609=DIRECTION('ref_axis',(-1.,0.,0.));
#27610=DIRECTION('',(0.,-1.,0.));
#27611=DIRECTION('',(0.,1.,0.));
#27612=DIRECTION('',(-1.,0.,0.));
#27613=DIRECTION('center_axis',(-1.,0.,0.));
#27614=DIRECTION('ref_axis',(0.,0.,1.));
#27615=DIRECTION('',(0.,0.,1.));
#27616=DIRECTION('center_axis',(0.,1.,0.));
#27617=DIRECTION('ref_axis',(0.,0.,1.));
#27618=DIRECTION('',(0.,0.,1.));
#27619=DIRECTION('center_axis',(1.,0.,0.));
#27620=DIRECTION('ref_axis',(0.,0.,-1.));
#34633=CARTESIAN_POINT('',(0.,0.,0.));
#34634=CARTESIAN_POINT('Origin',(-12.5,160.5,7.5));
#34635=CARTESIAN_POINT('',(-15.5,160.5,-7.5));
#34636=CARTESIAN_POINT('Origin',(-12.5,160.5,-7.5));
#34637=CARTESIAN_POINT('',(-15.5,160.5,7.5));
#34638=CARTESIAN_POINT('',(-15.5,160.5,7.5));
#34639=CARTESIAN_POINT('Origin',(-12.5,160.5,7.5));
#34640=CARTESIAN_POINT('Origin',(12.5,160.5,7.5));
#34641=CARTESIAN_POINT('',(9.50000000000003,160.5,-7.5));
#34642=CARTESIAN_POINT('Origin',(12.5,160.5,-7.5));
#34643=CARTESIAN_POINT('',(9.50000000000003,160.5,7.5));
#34644=CARTESIAN_POINT('',(9.50000000000003,160.5,7.5));
#34645=CARTESIAN_POINT('Origin',(12.5,160.5,7.5));
#34646=CARTESIAN_POINT('Origin',(-12.5,-190.,7.5));
#34647=CARTESIAN_POINT('',(-15.5,-190.,-7.5));
#34648=CARTESIAN_POINT('Origin',(-12.5,-190.,-7.5));
#34649=CARTESIAN_POINT('',(-15.5,-190.,7.5));
#34650=CARTESIAN_POINT('',(-15.5,-190.,7.5));
#34651=CARTESIAN_POINT('Origin',(-12.5,-190.,7.5));
#34652=CARTESIAN_POINT('Origin',(12.5,-190.,7.5));
#34653=CARTESIAN_POINT('',(9.50000000000003,-190.,-7.5));
#34654=CARTESIAN_POINT('Origin',(12.5,-190.,-7.5));
#34655=CARTESIAN_POINT('',(9.50000000000003,-190.,7.5));
#34656=CARTESIAN_POINT('',(9.50000000000003,-190.,7.5));
#34657=CARTESIAN_POINT('Origin',(12.5,-190.,7.5));
#34658=CARTESIAN_POINT('Origin',(-26.,160.5,7.5));
#34659=CARTESIAN_POINT('',(-29.4,160.5,-7.5));
#34660=CARTESIAN_POINT('Origin',(-26.,160.5,-7.5));
#34661=CARTESIAN_POINT('',(-29.4,160.5,7.5));
#34662=CARTESIAN_POINT('',(-29.4,160.5,7.5));
#34663=CARTESIAN_POINT('Origin',(-26.,160.5,7.5));
#34664=CARTESIAN_POINT('Origin',(26.,160.5,7.5));
#34665=CARTESIAN_POINT('',(22.6,160.5,-7.5));
#34666=CARTESIAN_POINT('Origin',(26.,160.5,-7.5));
#34667=CARTESIAN_POINT('',(22.6,160.5,7.5));
#34668=CARTESIAN_POINT('',(22.6,160.5,7.5));
#34669=CARTESIAN_POINT('Origin',(26.,160.5,7.5));
#34670=CARTESIAN_POINT('Origin',(-26.,-190.,7.5));
#34671=CARTESIAN_POINT('',(-29.4,-190.,-7.5));
#34672=CARTESIAN_POINT('Origin',(-26.,-190.,-7.5));
#34673=CARTESIAN_POINT('',(-29.4,-190.,7.5));
#34674=CARTESIAN_POINT('',(-29.4,-190.,7.5));
#34675=CARTESIAN_POINT('Origin',(-26.,-190.,7.5));
#34676=CARTESIAN_POINT('Origin',(26.,-190.,7.5));
#34677=CARTESIAN_POINT('',(22.6,-190.,-7.5));
#34678=CARTESIAN_POINT('Origin',(26.,-190.,-7.5));
#34679=CARTESIAN_POINT('',(22.6,-190.,7.5));
#34680=CARTESIAN_POINT('',(22.6,-190.,7.5));
#34681=CARTESIAN_POINT('Origin',(26.,-190.,7.5));
#34682=CARTESIAN_POINT('Origin',(-10.,260.,-6.93889390390723E-15));
#34683=CARTESIAN_POINT('',(-10.,250.,-3.));
#34684=CARTESIAN_POINT('Origin',(-10.,250.,-6.93889390390723E-15));
#34685=CARTESIAN_POINT('',(-10.,260.,-3.));
#34686=CARTESIAN_POINT('',(-10.,260.,-3.));
#34687=CARTESIAN_POINT('Origin',(-10.,260.,-6.93889390390723E-15));
#34688=CARTESIAN_POINT('Origin',(-10.,250.,-6.93889390390723E-15));
#34689=CARTESIAN_POINT('',(-10.,248.197418142917,-6.93889390390723E-15));
#34690=CARTESIAN_POINT('',(-10.,250.,-3.));
#34691=CARTESIAN_POINT('Origin',(10.,260.,-6.93889390390723E-15));
#34692=CARTESIAN_POINT('',(10.,250.,-3.));
#34693=CARTESIAN_POINT('Origin',(10.,250.,-6.93889390390723E-15));
#34694=CARTESIAN_POINT('',(10.,260.,-3.));
#34695=CARTESIAN_POINT('',(10.,260.,-3.));
#34696=CARTESIAN_POINT('Origin',(10.,260.,-6.93889390390723E-15));
#34697=CARTESIAN_POINT('Origin',(10.,250.,-6.93889390390723E-15));
#34698=CARTESIAN_POINT('',(9.99999999999999,248.197418142917,-6.93889390390723E-15));
#34699=CARTESIAN_POINT('',(10.,250.,-3.));
#34700=CARTESIAN_POINT('Origin',(-24.,260.,-6.93889390390723E-15));
#34701=CARTESIAN_POINT('',(-24.,243.,-2.5));
#34702=CARTESIAN_POINT('Origin',(-24.,243.,-6.93889390390723E-15));
#34703=CARTESIAN_POINT('',(-24.,260.,-2.5));
#34704=CARTESIAN_POINT('',(-24.,260.,-2.5));
#34705=CARTESIAN_POINT('Origin',(-24.,260.,-6.93889390390723E-15));
#34706=CARTESIAN_POINT('Origin',(-24.,243.,-6.93889390390723E-15));
#34707=CARTESIAN_POINT('',(-24.,241.497848452431,-6.93889390390723E-15));
#34708=CARTESIAN_POINT('',(-24.,243.,-2.5));
#34709=CARTESIAN_POINT('Origin',(24.,260.,-6.93889390390723E-15));
#34710=CARTESIAN_POINT('',(24.,243.,-2.5));
#34711=CARTESIAN_POINT('Origin',(24.,243.,-6.93889390390723E-15));
#34712=CARTESIAN_POINT('',(24.,260.,-2.5));
#34713=CARTESIAN_POINT('',(24.,260.,-2.5));
#34714=CARTESIAN_POINT('Origin',(24.,260.,-6.93889390390723E-15));
#34715=CARTESIAN_POINT('Origin',(24.,243.,-6.93889390390723E-15));
#34716=CARTESIAN_POINT('',(24.,241.497848452431,-6.93889390390723E-15));
#34717=CARTESIAN_POINT('',(24.,243.,-2.5));
#34718=CARTESIAN_POINT('Origin',(-150.,-260.,7.5));
#34719=CARTESIAN_POINT('',(-150.,-260.,-7.5));
#34720=CARTESIAN_POINT('',(-90.,-260.,-7.5));
#34721=CARTESIAN_POINT('',(-150.,-260.,-7.5));
#34722=CARTESIAN_POINT('',(-90.,-260.,7.5));
#34723=CARTESIAN_POINT('',(-90.,-260.,-7.5));
#34724=CARTESIAN_POINT('',(-150.,-260.,7.5));
#34725=CARTESIAN_POINT('',(-150.,-260.,7.5));
#34726=CARTESIAN_POINT('',(-150.,-260.,7.5));
#34727=CARTESIAN_POINT('Origin',(150.,-260.,7.5));
#34728=CARTESIAN_POINT('',(150.,-260.,-7.5));
#34729=CARTESIAN_POINT('',(150.,260.,-7.5));
#34730=CARTESIAN_POINT('',(150.,-260.,-7.5));
#34731=CARTESIAN_POINT('',(150.,260.,7.5));
#34732=CARTESIAN_POINT('',(150.,260.,7.5));
#34733=CARTESIAN_POINT('',(150.,-260.,7.5));
#34734=CARTESIAN_POINT('',(150.,-260.,7.5));
#34735=CARTESIAN_POINT('',(150.,-260.,7.5));
#34736=CARTESIAN_POINT('Origin',(-150.,260.,7.5));
#34737=CARTESIAN_POINT('',(-150.,260.,-7.5));
#34738=CARTESIAN_POINT('',(-150.,260.,-7.5));
#34739=CARTESIAN_POINT('',(-150.,260.,7.5));
#34740=CARTESIAN_POINT('',(-150.,260.,7.5));
#34741=CARTESIAN_POINT('',(-150.,260.,7.5));
#34742=CARTESIAN_POINT('Origin',(-150.,-260.,7.5));
#34743=CARTESIAN_POINT('',(-150.,-260.,-7.5));
#34744=CARTESIAN_POINT('',(-150.,-260.,7.5));
#34745=CARTESIAN_POINT('Origin',(-150.,-260.,7.5));
#34746=CARTESIAN_POINT('',(90.,-260.,7.5));
#34747=CARTESIAN_POINT('',(-150.,-260.,7.5));
#34748=CARTESIAN_POINT('',(90.,-260.,-7.5));
#34749=CARTESIAN_POINT('',(90.,-260.,-7.5));
#34750=CARTESIAN_POINT('',(-150.,-260.,-7.5));
#34751=CARTESIAN_POINT('Origin',(0.,0.,7.5));
#34752=CARTESIAN_POINT('',(-90.,-210.,7.5));
#34753=CARTESIAN_POINT('',(-90.,-210.,7.5));
#34754=CARTESIAN_POINT('',(90.,-210.,7.5));
#34755=CARTESIAN_POINT('',(-90.,-210.,7.5));
#34756=CARTESIAN_POINT('',(90.,-210.,7.5));
#34757=CARTESIAN_POINT('Origin',(0.,0.,-7.5));
#34758=CARTESIAN_POINT('',(-90.,-210.,-7.5));
#34759=CARTESIAN_POINT('',(-90.,-210.,-7.5));
#34760=CARTESIAN_POINT('',(90.,-210.,-7.5));
#34761=CARTESIAN_POINT('',(90.,-210.,-7.5));
#34762=CARTESIAN_POINT('',(-90.,-210.,-7.5));
#34763=CARTESIAN_POINT('Origin',(-90.,-210.,-7.5));
#34764=CARTESIAN_POINT('',(-90.,-210.,-7.5));
#34765=CARTESIAN_POINT('Origin',(-90.,-210.,-7.5));
#34766=CARTESIAN_POINT('',(90.,-210.,-7.5));
#34767=CARTESIAN_POINT('Origin',(90.,-210.,-7.5));
#57003=UNCERTAINTY_MEASURE_WITH_UNIT(LENGTH_MEASURE(0.01),#57080,
'DISTANCE_ACCURACY_VALUE',
'Maximum model space distance between geometric entities at asserted c
onnectivities');
#57040=UNCERTAINTY_MEASURE_WITH_UNIT(LENGTH_MEASURE(0.01),#57080,
'DISTANCE_ACCURACY_VALUE',
'Maximum model space distance between geometric entities at asserted c
onnectivities');
#57042=(
GEOMETRIC_REPRESENTATION_CONTEXT(3)
GLOBAL_UNCERTAINTY_ASSIGNED_CONTEXT((#57003))
GLOBAL_UNIT_ASSIGNED_CONTEXT((#57080,#57082,#57083))
REPRESENTATION_CONTEXT('','3D')
);
#57079=(
GEOMETRIC_REPRESENTATION_CONTEXT(3)
GLOBAL_UNCERTAINTY_ASSIGNED_CONTEXT((#57040))
GLOBAL_UNIT_ASSIGNED_CONTEXT((#57080,#57082,#57083))
REPRESENTATION_CONTEXT('','3D')
);
#57080=(
LENGTH_UNIT()
NAMED_UNIT(*)
SI_UNIT(.MILLI.,.METRE.)
);
#57082=(
NAMED_UNIT(*)
PLANE_ANGLE_UNIT()
SI_UNIT($,.RADIAN.)
);
#57083=(
NAMED_UNIT(*)
SI_UNIT($,.STERADIAN.)
SOLID_ANGLE_UNIT()
);
#57085=SHAPE_DEFINITION_REPRESENTATION(#57123,#57250);
#57123=PRODUCT_DEFINITION_SHAPE('',$,#57289);
#57250=SHAPE_REPRESENTATION('',(#24884),#57042);
#57287=PRODUCT_DEFINITION_CONTEXT('part definition',#57403,'design');
#57289=PRODUCT_DEFINITION('Main Plate','Main Plate',#57327,#57287);
#57327=PRODUCT_DEFINITION_FORMATION('',$,#57406);
#57403=APPLICATION_CONTEXT(
'Core Data for Automotive Mechanical Design Process');
#57404=PRODUCT_CONTEXT('part definition',#57403,'mechanical');
#57406=PRODUCT('Main Plate','Main Plate',$,(#57404));
#57444=PRESENTATION_STYLE_ASSIGNMENT((#57446));
#57446=SURFACE_STYLE_USAGE(.BOTH.,#57448);
#57448=SURFACE_SIDE_STYLE('',(#57450));
#57450=SURFACE_STYLE_FILL_AREA(#57452);
#57452=FILL_AREA_STYLE('Opaque(202,209,238)',(#57454));
#57454=FILL_AREA_STYLE_COLOUR('Opaque(202,209,238)',#57456);
#57456=COLOUR_RGB('Opaque(202,209,238)',0.792156862745098,0.819607843137255,
0.933333333333333);
ENDSEC;
END-ISO-10303-21;
